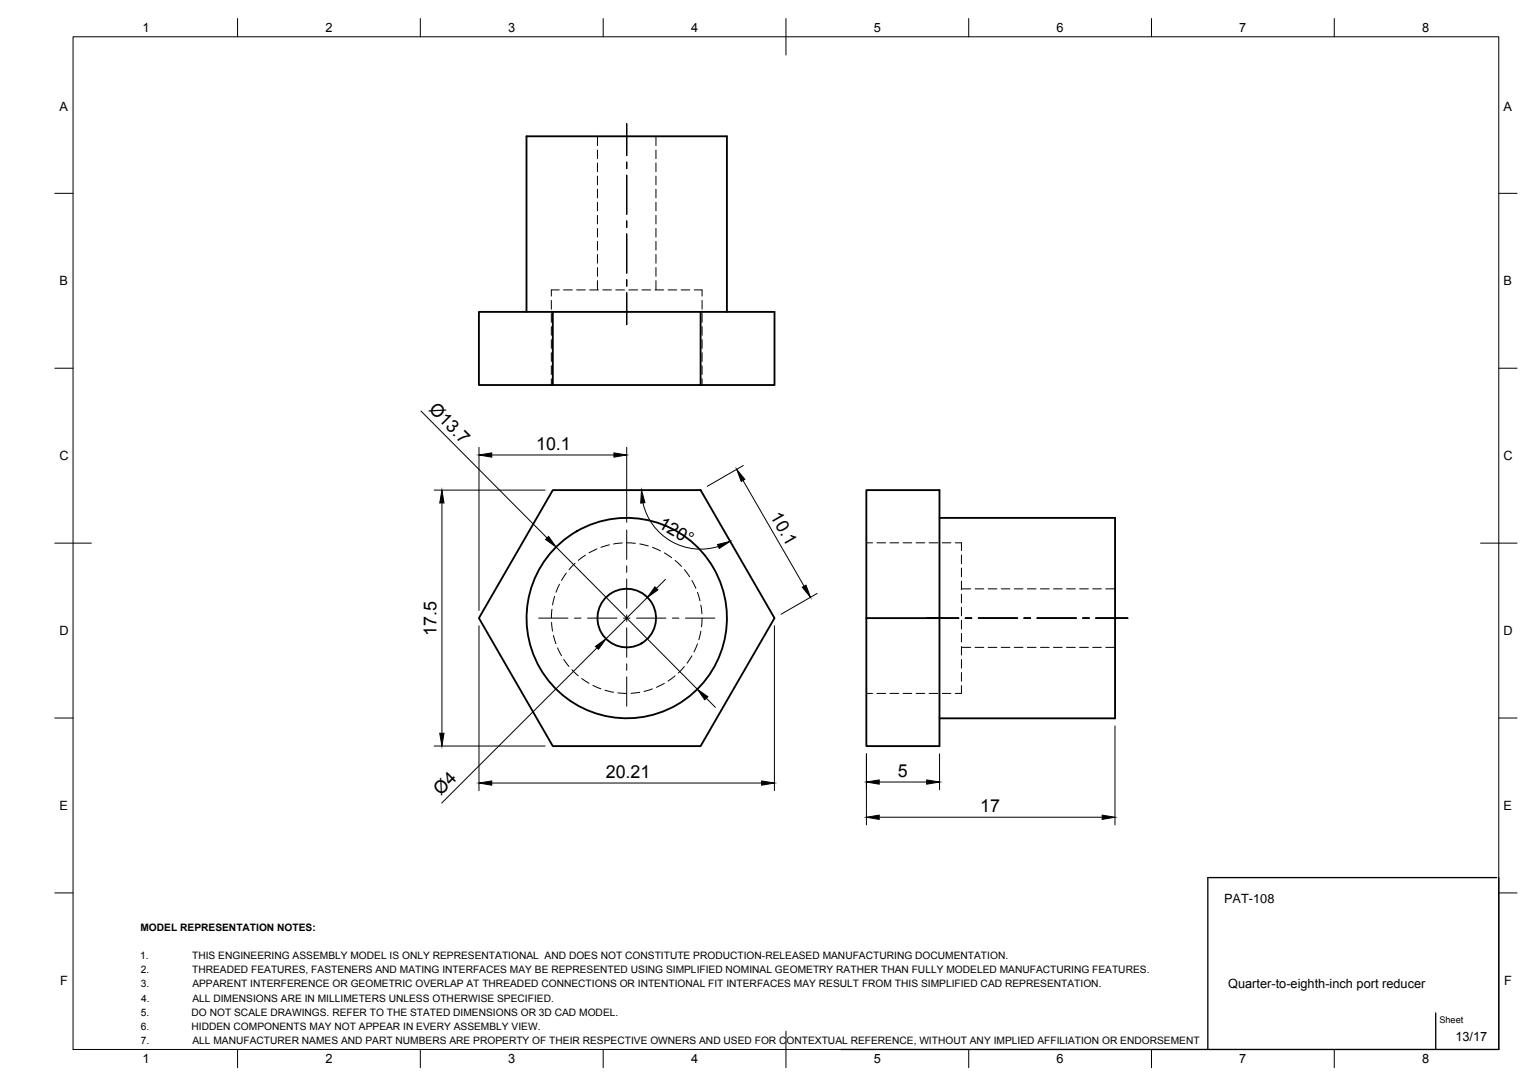
ISO-10303-21;
HEADER;
/* Generated by software containing ST-Developer
 * from STEP Tools, Inc. (www.steptools.com) 
 */

FILE_DESCRIPTION(
/* description */ ('Sub-base valve envelopes and connections'),
/* implementation_level */ '2;1');

FILE_NAME(
/* name */ 'Quarter-to-eighth-inch port reducer.step',
/* time_stamp */ '2026-10-29T15:55:44-07:00',
/* author */ (''),
/* organization */ (''),
/* preprocessor_version */ 'ST-DEVELOPER v20.2',
/* originating_system */ 'Autodesk Translation Framework v15.17.0.0',
/* authorisation */ '');

FILE_SCHEMA (('AUTOMOTIVE_DESIGN { 1 0 10303 214 3 1 1 }'));
ENDSEC;

DATA;
#10=MECHANICAL_DESIGN_GEOMETRIC_PRESENTATION_REPRESENTATION('',(#127),#6113);
#103=SHAPE_REPRESENTATION_RELATIONSHIP('SRR','None',#6177,#115);
#115=ADVANCED_BREP_SHAPE_REPRESENTATION('',(#139),#6108);
#127=STYLED_ITEM('',(#6301),#139);
#139=MANIFOLD_SOLID_BREP('Body1',#3366);
#245=FACE_BOUND('',#836,.T.);
#246=FACE_BOUND('',#838,.T.);
#247=FACE_BOUND('',#846,.T.);
#248=FACE_BOUND('',#850,.T.);
#350=PLANE('',#3802);
#351=PLANE('',#3804);
#352=PLANE('',#3806);
#353=PLANE('',#3807);
#354=PLANE('',#3808);
#355=PLANE('',#3809);
#356=PLANE('',#3810);
#357=PLANE('',#3811);
#358=PLANE('',#3812);
#359=PLANE('',#3817);
#532=FACE_OUTER_BOUND('',#834,.T.);
#533=FACE_OUTER_BOUND('',#835,.T.);
#534=FACE_OUTER_BOUND('',#837,.T.);
#535=FACE_OUTER_BOUND('',#839,.T.);
#536=FACE_OUTER_BOUND('',#840,.T.);
#537=FACE_OUTER_BOUND('',#841,.T.);
#538=FACE_OUTER_BOUND('',#842,.T.);
#539=FACE_OUTER_BOUND('',#843,.T.);
#540=FACE_OUTER_BOUND('',#844,.T.);
#541=FACE_OUTER_BOUND('',#845,.T.);
#542=FACE_OUTER_BOUND('',#847,.T.);
#543=FACE_OUTER_BOUND('',#848,.T.);
#544=FACE_OUTER_BOUND('',#849,.T.);
#834=EDGE_LOOP('',(#2873,#2874,#2875,#2876));
#835=EDGE_LOOP('',(#2877));
#836=EDGE_LOOP('',(#2878));
#837=EDGE_LOOP('',(#2879,#2880,#2881,#2882,#2883,#2884));
#838=EDGE_LOOP('',(#2885));
#839=EDGE_LOOP('',(#2886,#2887,#2888,#2889));
#840=EDGE_LOOP('',(#2890,#2891,#2892,#2893));
#841=EDGE_LOOP('',(#2894,#2895,#2896,#2897));
#842=EDGE_LOOP('',(#2898,#2899,#2900,#2901));
#843=EDGE_LOOP('',(#2902,#2903,#2904,#2905));
#844=EDGE_LOOP('',(#2906,#2907,#2908,#2909));
#845=EDGE_LOOP('',(#2910,#2911,#2912,#2913,#2914,#2915));
#846=EDGE_LOOP('',(#2916));
#847=EDGE_LOOP('',(#2917,#2918,#2919,#2920));
#848=EDGE_LOOP('',(#2921,#2922,#2923,#2924));
#849=EDGE_LOOP('',(#2925));
#850=EDGE_LOOP('',(#2926));
#1064=LINE('',#5843,#1298);
#1065=LINE('',#5851,#1299);
#1066=LINE('',#5853,#1300);
#1067=LINE('',#5855,#1301);
#1068=LINE('',#5857,#1302);
#1069=LINE('',#5859,#1303);
#1070=LINE('',#5860,#1304);
#1071=LINE('',#5865,#1305);
#1072=LINE('',#5867,#1306);
#1073=LINE('',#5868,#1307);
#1074=LINE('',#5871,#1308);
#1075=LINE('',#5872,#1309);
#1076=LINE('',#5875,#1310);
#1077=LINE('',#5876,#1311);
#1078=LINE('',#5879,#1312);
#1079=LINE('',#5880,#1313);
#1080=LINE('',#5883,#1314);
#1081=LINE('',#5884,#1315);
#1082=LINE('',#5886,#1316);
#1083=LINE('',#5890,#1317);
#1084=LINE('',#5894,#1318);
#1298=VECTOR('',#4662,0.515);
#1299=VECTOR('',#4671,1.);
#1300=VECTOR('',#4672,1.);
#1301=VECTOR('',#4673,1.);
#1302=VECTOR('',#4674,1.);
#1303=VECTOR('',#4675,1.);
#1304=VECTOR('',#4676,1.);
#1305=VECTOR('',#4681,1.);
#1306=VECTOR('',#4682,1.);
#1307=VECTOR('',#4683,1.);
#1308=VECTOR('',#4686,1.);
#1309=VECTOR('',#4687,1.);
#1310=VECTOR('',#4690,1.);
#1311=VECTOR('',#4691,1.);
#1312=VECTOR('',#4694,1.);
#1313=VECTOR('',#4695,1.);
#1314=VECTOR('',#4698,1.);
#1315=VECTOR('',#4699,1.);
#1316=VECTOR('',#4702,1.);
#1317=VECTOR('',#4707,0.2);
#1318=VECTOR('',#4712,0.685);
#1507=CIRCLE('',#3800,0.515);
#1508=CIRCLE('',#3801,0.515);
#1509=CIRCLE('',#3803,0.2);
#1510=CIRCLE('',#3805,0.685);
#1511=CIRCLE('',#3814,0.2);
#1512=CIRCLE('',#3816,0.685);
#1749=VERTEX_POINT('',#5840);
#1750=VERTEX_POINT('',#5842);
#1751=VERTEX_POINT('',#5846);
#1752=VERTEX_POINT('',#5849);
#1753=VERTEX_POINT('',#5850);
#1754=VERTEX_POINT('',#5852);
#1755=VERTEX_POINT('',#5854);
#1756=VERTEX_POINT('',#5856);
#1757=VERTEX_POINT('',#5858);
#1758=VERTEX_POINT('',#5861);
#1759=VERTEX_POINT('',#5864);
#1760=VERTEX_POINT('',#5866);
#1761=VERTEX_POINT('',#5870);
#1762=VERTEX_POINT('',#5874);
#1763=VERTEX_POINT('',#5878);
#1764=VERTEX_POINT('',#5882);
#1765=VERTEX_POINT('',#5889);
#1766=VERTEX_POINT('',#5893);
#2134=EDGE_CURVE('',#1749,#1749,#1507,.T.);
#2135=EDGE_CURVE('',#1749,#1750,#1064,.T.);
#2136=EDGE_CURVE('',#1750,#1750,#1508,.T.);
#2137=EDGE_CURVE('',#1751,#1751,#1509,.T.);
#2138=EDGE_CURVE('',#1752,#1753,#1065,.T.);
#2139=EDGE_CURVE('',#1754,#1752,#1066,.T.);
#2140=EDGE_CURVE('',#1755,#1754,#1067,.T.);
#2141=EDGE_CURVE('',#1756,#1755,#1068,.T.);
#2142=EDGE_CURVE('',#1757,#1756,#1069,.T.);
#2143=EDGE_CURVE('',#1753,#1757,#1070,.T.);
#2144=EDGE_CURVE('',#1758,#1758,#1510,.T.);
#2145=EDGE_CURVE('',#1752,#1759,#1071,.T.);
#2146=EDGE_CURVE('',#1760,#1759,#1072,.T.);
#2147=EDGE_CURVE('',#1754,#1760,#1073,.T.);
#2148=EDGE_CURVE('',#1761,#1760,#1074,.T.);
#2149=EDGE_CURVE('',#1755,#1761,#1075,.T.);
#2150=EDGE_CURVE('',#1762,#1761,#1076,.T.);
#2151=EDGE_CURVE('',#1756,#1762,#1077,.T.);
#2152=EDGE_CURVE('',#1763,#1762,#1078,.T.);
#2153=EDGE_CURVE('',#1757,#1763,#1079,.T.);
#2154=EDGE_CURVE('',#1764,#1763,#1080,.T.);
#2155=EDGE_CURVE('',#1753,#1764,#1081,.T.);
#2156=EDGE_CURVE('',#1759,#1764,#1082,.T.);
#2157=EDGE_CURVE('',#1751,#1765,#1083,.T.);
#2158=EDGE_CURVE('',#1765,#1765,#1511,.T.);
#2159=EDGE_CURVE('',#1758,#1766,#1084,.T.);
#2160=EDGE_CURVE('',#1766,#1766,#1512,.T.);
#2873=ORIENTED_EDGE('',*,*,#2134,.F.);
#2874=ORIENTED_EDGE('',*,*,#2135,.T.);
#2875=ORIENTED_EDGE('',*,*,#2136,.F.);
#2876=ORIENTED_EDGE('',*,*,#2135,.F.);
#2877=ORIENTED_EDGE('',*,*,#2134,.T.);
#2878=ORIENTED_EDGE('',*,*,#2137,.F.);
#2879=ORIENTED_EDGE('',*,*,#2138,.F.);
#2880=ORIENTED_EDGE('',*,*,#2139,.F.);
#2881=ORIENTED_EDGE('',*,*,#2140,.F.);
#2882=ORIENTED_EDGE('',*,*,#2141,.F.);
#2883=ORIENTED_EDGE('',*,*,#2142,.F.);
#2884=ORIENTED_EDGE('',*,*,#2143,.F.);
#2885=ORIENTED_EDGE('',*,*,#2144,.T.);
#2886=ORIENTED_EDGE('',*,*,#2139,.T.);
#2887=ORIENTED_EDGE('',*,*,#2145,.T.);
#2888=ORIENTED_EDGE('',*,*,#2146,.F.);
#2889=ORIENTED_EDGE('',*,*,#2147,.F.);
#2890=ORIENTED_EDGE('',*,*,#2140,.T.);
#2891=ORIENTED_EDGE('',*,*,#2147,.T.);
#2892=ORIENTED_EDGE('',*,*,#2148,.F.);
#2893=ORIENTED_EDGE('',*,*,#2149,.F.);
#2894=ORIENTED_EDGE('',*,*,#2141,.T.);
#2895=ORIENTED_EDGE('',*,*,#2149,.T.);
#2896=ORIENTED_EDGE('',*,*,#2150,.F.);
#2897=ORIENTED_EDGE('',*,*,#2151,.F.);
#2898=ORIENTED_EDGE('',*,*,#2142,.T.);
#2899=ORIENTED_EDGE('',*,*,#2151,.T.);
#2900=ORIENTED_EDGE('',*,*,#2152,.F.);
#2901=ORIENTED_EDGE('',*,*,#2153,.F.);
#2902=ORIENTED_EDGE('',*,*,#2143,.T.);
#2903=ORIENTED_EDGE('',*,*,#2153,.T.);
#2904=ORIENTED_EDGE('',*,*,#2154,.F.);
#2905=ORIENTED_EDGE('',*,*,#2155,.F.);
#2906=ORIENTED_EDGE('',*,*,#2138,.T.);
#2907=ORIENTED_EDGE('',*,*,#2155,.T.);
#2908=ORIENTED_EDGE('',*,*,#2156,.F.);
#2909=ORIENTED_EDGE('',*,*,#2145,.F.);
#2910=ORIENTED_EDGE('',*,*,#2156,.T.);
#2911=ORIENTED_EDGE('',*,*,#2154,.T.);
#2912=ORIENTED_EDGE('',*,*,#2152,.T.);
#2913=ORIENTED_EDGE('',*,*,#2150,.T.);
#2914=ORIENTED_EDGE('',*,*,#2148,.T.);
#2915=ORIENTED_EDGE('',*,*,#2146,.T.);
#2916=ORIENTED_EDGE('',*,*,#2136,.T.);
#2917=ORIENTED_EDGE('',*,*,#2137,.T.);
#2918=ORIENTED_EDGE('',*,*,#2157,.T.);
#2919=ORIENTED_EDGE('',*,*,#2158,.T.);
#2920=ORIENTED_EDGE('',*,*,#2157,.F.);
#2921=ORIENTED_EDGE('',*,*,#2144,.F.);
#2922=ORIENTED_EDGE('',*,*,#2159,.T.);
#2923=ORIENTED_EDGE('',*,*,#2160,.T.);
#2924=ORIENTED_EDGE('',*,*,#2159,.F.);
#2925=ORIENTED_EDGE('',*,*,#2160,.F.);
#2926=ORIENTED_EDGE('',*,*,#2158,.F.);
#3146=CYLINDRICAL_SURFACE('',#3799,0.515);
#3147=CYLINDRICAL_SURFACE('',#3813,0.2);
#3148=CYLINDRICAL_SURFACE('',#3815,0.685);
#3305=ADVANCED_FACE('',(#532),#3146,.F.);
#3306=ADVANCED_FACE('',(#533,#245),#350,.T.);
#3307=ADVANCED_FACE('',(#534,#246),#351,.F.);
#3308=ADVANCED_FACE('',(#535),#352,.T.);
#3309=ADVANCED_FACE('',(#536),#353,.T.);
#3310=ADVANCED_FACE('',(#537),#354,.T.);
#3311=ADVANCED_FACE('',(#538),#355,.T.);
#3312=ADVANCED_FACE('',(#539),#356,.T.);
#3313=ADVANCED_FACE('',(#540),#357,.T.);
#3314=ADVANCED_FACE('',(#541,#247),#358,.T.);
#3315=ADVANCED_FACE('',(#542),#3147,.F.);
#3316=ADVANCED_FACE('',(#543),#3148,.T.);
#3317=ADVANCED_FACE('',(#544,#248),#359,.F.);
#3366=CLOSED_SHELL('',(#3305,#3306,#3307,#3308,#3309,#3310,#3311,#3312,
#3313,#3314,#3315,#3316,#3317));
#3798=AXIS2_PLACEMENT_3D('',#5838,#4656,#4657);
#3799=AXIS2_PLACEMENT_3D('',#5839,#4658,#4659);
#3800=AXIS2_PLACEMENT_3D('',#5841,#4660,#4661);
#3801=AXIS2_PLACEMENT_3D('',#5844,#4663,#4664);
#3802=AXIS2_PLACEMENT_3D('',#5845,#4665,#4666);
#3803=AXIS2_PLACEMENT_3D('',#5847,#4667,#4668);
#3804=AXIS2_PLACEMENT_3D('',#5848,#4669,#4670);
#3805=AXIS2_PLACEMENT_3D('',#5862,#4677,#4678);
#3806=AXIS2_PLACEMENT_3D('',#5863,#4679,#4680);
#3807=AXIS2_PLACEMENT_3D('',#5869,#4684,#4685);
#3808=AXIS2_PLACEMENT_3D('',#5873,#4688,#4689);
#3809=AXIS2_PLACEMENT_3D('',#5877,#4692,#4693);
#3810=AXIS2_PLACEMENT_3D('',#5881,#4696,#4697);
#3811=AXIS2_PLACEMENT_3D('',#5885,#4700,#4701);
#3812=AXIS2_PLACEMENT_3D('',#5887,#4703,#4704);
#3813=AXIS2_PLACEMENT_3D('',#5888,#4705,#4706);
#3814=AXIS2_PLACEMENT_3D('',#5891,#4708,#4709);
#3815=AXIS2_PLACEMENT_3D('',#5892,#4710,#4711);
#3816=AXIS2_PLACEMENT_3D('',#5895,#4713,#4714);
#3817=AXIS2_PLACEMENT_3D('',#5896,#4715,#4716);
#4656=DIRECTION('axis',(0.,0.,1.));
#4657=DIRECTION('refdir',(1.,0.,0.));
#4658=DIRECTION('center_axis',(0.,0.,1.));
#4659=DIRECTION('ref_axis',(1.,0.,0.));
#4660=DIRECTION('center_axis',(0.,0.,1.));
#4661=DIRECTION('ref_axis',(1.,0.,0.));
#4662=DIRECTION('',(0.,0.,1.));
#4663=DIRECTION('center_axis',(0.,0.,-1.));
#4664=DIRECTION('ref_axis',(1.,0.,0.));
#4665=DIRECTION('center_axis',(0.,0.,1.));
#4666=DIRECTION('ref_axis',(1.,0.,0.));
#4667=DIRECTION('center_axis',(0.,0.,1.));
#4668=DIRECTION('ref_axis',(1.,0.,0.));
#4669=DIRECTION('center_axis',(0.,0.,1.));
#4670=DIRECTION('ref_axis',(1.,0.,0.));
#4671=DIRECTION('',(0.5,0.866025403784438,0.));
#4672=DIRECTION('',(1.,-3.29650746237182E-16,0.));
#4673=DIRECTION('',(0.499999999999999,-0.866025403784439,0.));
#4674=DIRECTION('',(-0.5,-0.866025403784439,0.));
#4675=DIRECTION('',(-1.,0.,0.));
#4676=DIRECTION('',(-0.5,0.866025403784438,0.));
#4677=DIRECTION('center_axis',(0.,0.,1.));
#4678=DIRECTION('ref_axis',(1.,0.,0.));
#4679=DIRECTION('center_axis',(-3.29650746237182E-16,-1.,0.));
#4680=DIRECTION('ref_axis',(1.,-3.29650746237182E-16,0.));
#4681=DIRECTION('',(0.,0.,1.));
#4682=DIRECTION('',(1.,-3.29650746237182E-16,0.));
#4683=DIRECTION('',(0.,0.,1.));
#4684=DIRECTION('center_axis',(-0.866025403784439,-0.499999999999999,0.));
#4685=DIRECTION('ref_axis',(0.499999999999999,-0.866025403784439,0.));
#4686=DIRECTION('',(0.499999999999999,-0.866025403784439,0.));
#4687=DIRECTION('',(0.,0.,1.));
#4688=DIRECTION('center_axis',(-0.866025403784439,0.5,0.));
#4689=DIRECTION('ref_axis',(-0.5,-0.866025403784439,0.));
#4690=DIRECTION('',(-0.5,-0.866025403784439,0.));
#4691=DIRECTION('',(0.,0.,1.));
#4692=DIRECTION('center_axis',(0.,1.,0.));
#4693=DIRECTION('ref_axis',(-1.,0.,0.));
#4694=DIRECTION('',(-1.,0.,0.));
#4695=DIRECTION('',(0.,0.,1.));
#4696=DIRECTION('center_axis',(0.866025403784438,0.5,0.));
#4697=DIRECTION('ref_axis',(-0.5,0.866025403784438,0.));
#4698=DIRECTION('',(-0.5,0.866025403784438,0.));
#4699=DIRECTION('',(0.,0.,1.));
#4700=DIRECTION('center_axis',(0.866025403784438,-0.5,0.));
#4701=DIRECTION('ref_axis',(0.5,0.866025403784438,0.));
#4702=DIRECTION('',(0.5,0.866025403784438,0.));
#4703=DIRECTION('center_axis',(0.,0.,1.));
#4704=DIRECTION('ref_axis',(1.,0.,0.));
#4705=DIRECTION('center_axis',(0.,0.,1.));
#4706=DIRECTION('ref_axis',(1.,0.,0.));
#4707=DIRECTION('',(0.,0.,-1.));
#4708=DIRECTION('center_axis',(0.,0.,-1.));
#4709=DIRECTION('ref_axis',(1.,0.,0.));
#4710=DIRECTION('center_axis',(0.,0.,1.));
#4711=DIRECTION('ref_axis',(1.,0.,0.));
#4712=DIRECTION('',(0.,0.,-1.));
#4713=DIRECTION('center_axis',(0.,0.,1.));
#4714=DIRECTION('ref_axis',(1.,0.,0.));
#4715=DIRECTION('center_axis',(0.,0.,1.));
#4716=DIRECTION('ref_axis',(1.,0.,0.));
#5838=CARTESIAN_POINT('',(0.,0.,0.));
#5839=CARTESIAN_POINT('Origin',(-3.75,0.,4.85));
#5840=CARTESIAN_POINT('',(-4.265,-6.30693101560887E-17,4.85));
#5841=CARTESIAN_POINT('Origin',(-3.75,0.,4.85));
#5842=CARTESIAN_POINT('',(-4.265,6.30693101560887E-17,5.5));
#5843=CARTESIAN_POINT('',(-4.265,-6.30693101560887E-17,4.85));
#5844=CARTESIAN_POINT('Origin',(-3.75,0.,5.5));
#5845=CARTESIAN_POINT('Origin',(-3.75,0.,4.85));
#5846=CARTESIAN_POINT('',(-3.95,-2.44929359829471E-17,4.85));
#5847=CARTESIAN_POINT('Origin',(-3.75,0.,4.85));
#5848=CARTESIAN_POINT('Origin',(-3.75,0.,5.));
#5849=CARTESIAN_POINT('',(-3.24481851445908,-0.875,5.));
#5850=CARTESIAN_POINT('',(-2.73963702891815,0.,5.));
#5851=CARTESIAN_POINT('',(-3.24481851445908,-0.875,5.));
#5852=CARTESIAN_POINT('',(-4.25518148554092,-0.875,5.));
#5853=CARTESIAN_POINT('',(-4.25518148554092,-0.875,5.));
#5854=CARTESIAN_POINT('',(-4.76036297108184,1.23733777851239E-16,5.));
#5855=CARTESIAN_POINT('',(-4.76036297108184,1.23733777851239E-16,5.));
#5856=CARTESIAN_POINT('',(-4.25518148554092,0.875,5.));
#5857=CARTESIAN_POINT('',(-4.25518148554092,0.875,5.));
#5858=CARTESIAN_POINT('',(-3.24481851445908,0.875,5.));
#5859=CARTESIAN_POINT('',(-3.24481851445908,0.875,5.));
#5860=CARTESIAN_POINT('',(-2.73963702891815,0.,5.));
#5861=CARTESIAN_POINT('',(-4.435,-8.38883057415937E-17,5.));
#5862=CARTESIAN_POINT('Origin',(-3.75,0.,5.));
#5863=CARTESIAN_POINT('Origin',(-4.25518148554092,-0.875,5.));
#5864=CARTESIAN_POINT('',(-3.24481851445908,-0.875,5.5));
#5865=CARTESIAN_POINT('',(-3.24481851445908,-0.875,5.));
#5866=CARTESIAN_POINT('',(-4.25518148554092,-0.875,5.5));
#5867=CARTESIAN_POINT('',(-4.25518148554092,-0.875,5.5));
#5868=CARTESIAN_POINT('',(-4.25518148554092,-0.875,5.));
#5869=CARTESIAN_POINT('Origin',(-4.76036297108184,1.23733777851239E-16,
5.));
#5870=CARTESIAN_POINT('',(-4.76036297108184,1.11022302462516E-16,5.5));
#5871=CARTESIAN_POINT('',(-4.76036297108184,1.23733777851239E-16,5.5));
#5872=CARTESIAN_POINT('',(-4.76036297108184,1.23733777851239E-16,5.));
#5873=CARTESIAN_POINT('Origin',(-4.25518148554092,0.875,5.));
#5874=CARTESIAN_POINT('',(-4.25518148554092,0.875,5.5));
#5875=CARTESIAN_POINT('',(-4.25518148554092,0.875,5.5));
#5876=CARTESIAN_POINT('',(-4.25518148554092,0.875,5.));
#5877=CARTESIAN_POINT('Origin',(-3.24481851445908,0.875,5.));
#5878=CARTESIAN_POINT('',(-3.24481851445908,0.875,5.5));
#5879=CARTESIAN_POINT('',(-3.24481851445908,0.875,5.5));
#5880=CARTESIAN_POINT('',(-3.24481851445908,0.875,5.));
#5881=CARTESIAN_POINT('Origin',(-2.73963702891815,0.,5.));
#5882=CARTESIAN_POINT('',(-2.73963702891815,0.,5.5));
#5883=CARTESIAN_POINT('',(-2.73963702891815,0.,5.5));
#5884=CARTESIAN_POINT('',(-2.73963702891815,0.,5.));
#5885=CARTESIAN_POINT('Origin',(-3.24481851445908,-0.875,5.));
#5886=CARTESIAN_POINT('',(-3.24481851445908,-0.875,5.5));
#5887=CARTESIAN_POINT('Origin',(-3.75,0.,5.5));
#5888=CARTESIAN_POINT('Origin',(-3.75,0.,3.8));
#5889=CARTESIAN_POINT('',(-3.95,-2.44929359829471E-17,3.8));
#5890=CARTESIAN_POINT('',(-3.95,-2.44929359829471E-17,3.8));
#5891=CARTESIAN_POINT('Origin',(-3.75,0.,3.8));
#5892=CARTESIAN_POINT('Origin',(-3.75,0.,3.8));
#5893=CARTESIAN_POINT('',(-4.435,-8.38883057415937E-17,3.8));
#5894=CARTESIAN_POINT('',(-4.435,-8.38883057415937E-17,3.8));
#5895=CARTESIAN_POINT('Origin',(-3.75,0.,3.8));
#5896=CARTESIAN_POINT('Origin',(-3.75,0.,3.8));
#6092=UNCERTAINTY_MEASURE_WITH_UNIT(LENGTH_MEASURE(0.001),#6114,
'DISTANCE_ACCURACY_VALUE',
'Maximum model space distance between geometric entities at asserted c
onnectivities');
#6097=UNCERTAINTY_MEASURE_WITH_UNIT(LENGTH_MEASURE(0.001),#6114,
'DISTANCE_ACCURACY_VALUE',
'Maximum model space distance between geometric entities at asserted c
onnectivities');
#6108=(
GEOMETRIC_REPRESENTATION_CONTEXT(3)
GLOBAL_UNCERTAINTY_ASSIGNED_CONTEXT((#6092))
GLOBAL_UNIT_ASSIGNED_CONTEXT((#6114,#6116,#6117))
REPRESENTATION_CONTEXT('','3D')
);
#6113=(
GEOMETRIC_REPRESENTATION_CONTEXT(3)
GLOBAL_UNCERTAINTY_ASSIGNED_CONTEXT((#6097))
GLOBAL_UNIT_ASSIGNED_CONTEXT((#6114,#6116,#6117))
REPRESENTATION_CONTEXT('','3D')
);
#6114=(
LENGTH_UNIT()
NAMED_UNIT(*)
SI_UNIT(.CENTI.,.METRE.)
);
#6116=(
NAMED_UNIT(*)
PLANE_ANGLE_UNIT()
SI_UNIT($,.RADIAN.)
);
#6117=(
NAMED_UNIT(*)
SI_UNIT($,.STERADIAN.)
SOLID_ANGLE_UNIT()
);
#6128=SHAPE_DEFINITION_REPRESENTATION(#6143,#6177);
#6143=PRODUCT_DEFINITION_SHAPE('',$,#6193);
#6177=SHAPE_REPRESENTATION('',(#3798),#6108);
#6182=PRODUCT_DEFINITION_CONTEXT('part definition',#6229,'design');
#6193=PRODUCT_DEFINITION('Quarter-to-eighth-inch port reducer',
'Quarter-to-eighth-inch port reducer',#6208,#6182);
#6208=PRODUCT_DEFINITION_FORMATION('',$,#6241);
#6229=APPLICATION_CONTEXT(
'Core Data for Automotive Mechanical Design Process');
#6230=PRODUCT_CONTEXT('part definition',#6229,'mechanical');
#6241=PRODUCT('Quarter-to-eighth-inch port reducer',
'Quarter-to-eighth-inch port reducer',
'Quarter-to-eighth-inch port reducer',(#6230));
#6295=COLOUR_RGB('Light Blue',0.38,0.62,0.78);
#6296=FILL_AREA_STYLE_COLOUR('',#6295);
#6297=FILL_AREA_STYLE('',(#6296));
#6298=SURFACE_STYLE_FILL_AREA(#6297);
#6299=SURFACE_SIDE_STYLE('',(#6298));
#6300=SURFACE_STYLE_USAGE(.BOTH.,#6299);
#6301=PRESENTATION_STYLE_ASSIGNMENT((#6300));
ENDSEC;
END-ISO-10303-21;
